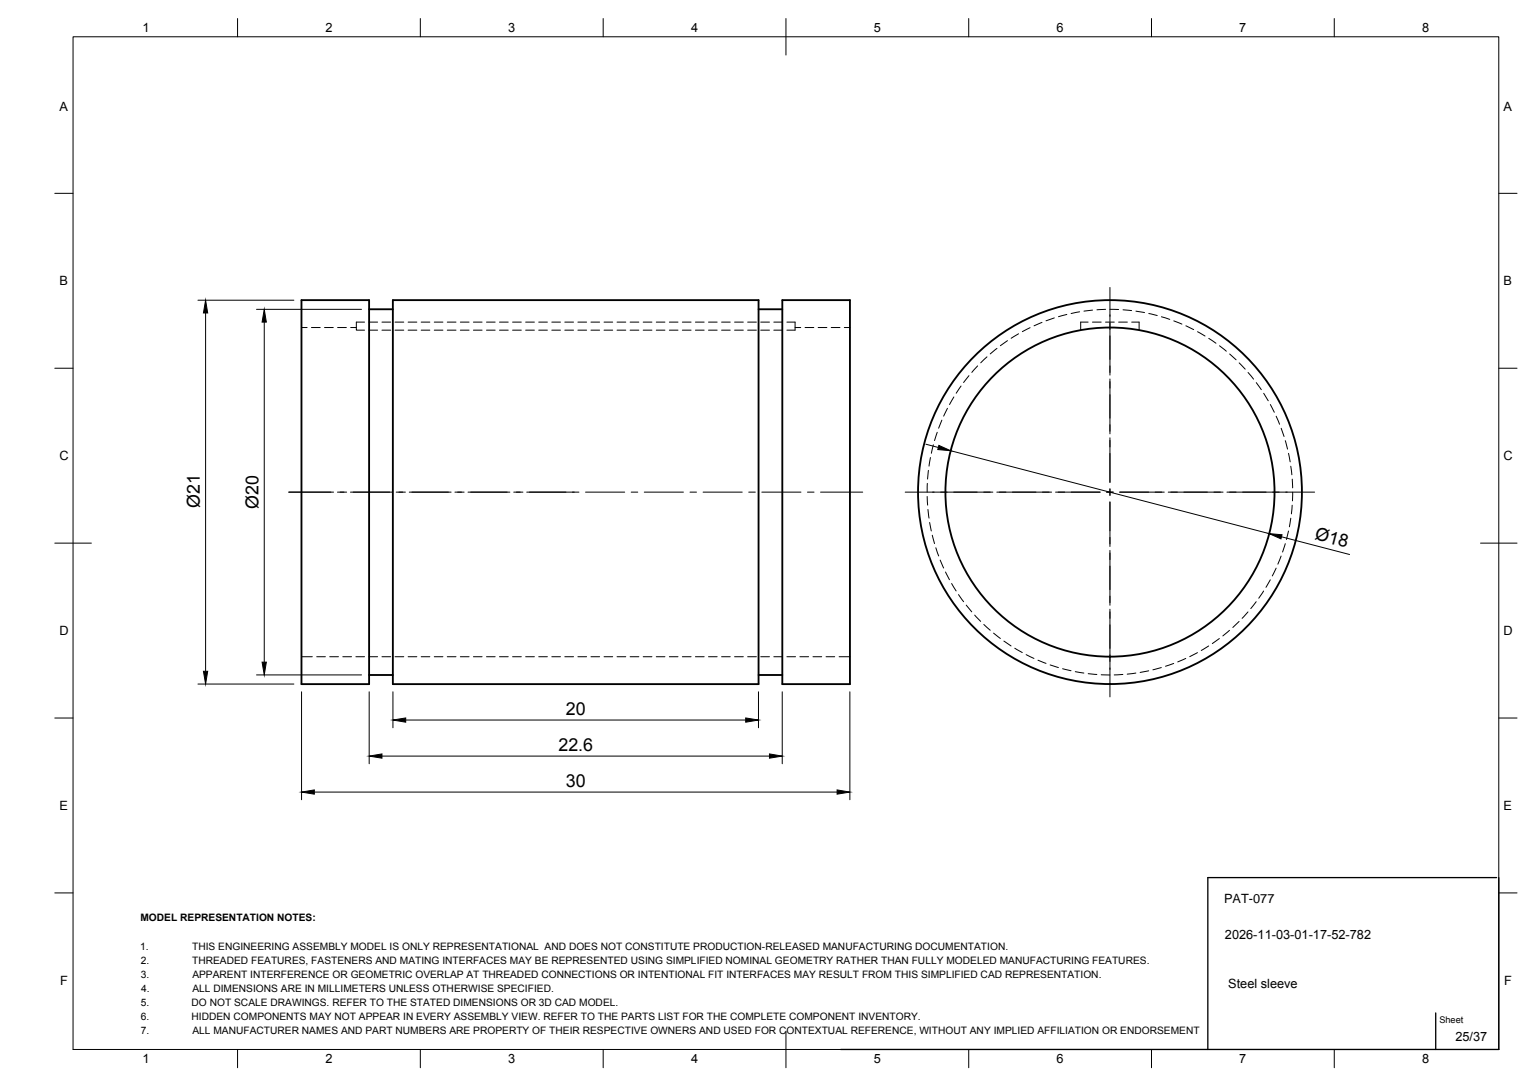
ISO-10303-21;
HEADER;
/* Generated by software containing ST-Developer
 * from STEP Tools, Inc. (www.steptools.com) 
 */

FILE_DESCRIPTION(
/* description */ ('Pallet stop with pneumatic fitting'),
/* implementation_level */ '2;1');

FILE_NAME(
/* name */ 'Steel sleeve.step',
/* time_stamp */ '2026-10-27T10:51:41-07:00',
/* author */ (''),
/* organization */ (''),
/* preprocessor_version */ 'ST-DEVELOPER v20.2',
/* originating_system */ 'Autodesk Translation Framework v15.17.0.0',
/* authorisation */ '');

FILE_SCHEMA (('AUTOMOTIVE_DESIGN { 1 0 10303 214 3 1 1 }'));
ENDSEC;

DATA;
#10=MECHANICAL_DESIGN_GEOMETRIC_PRESENTATION_REPRESENTATION('',(#375),#10265);
#311=SHAPE_REPRESENTATION_RELATIONSHIP('SRR','None',#10425,#343);
#343=ADVANCED_BREP_SHAPE_REPRESENTATION('',(#407),#10249);
#375=STYLED_ITEM('',(#10669),#407);
#407=MANIFOLD_SOLID_BREP('Body1',#5063);
#504=FACE_BOUND('',#1299,.T.);
#505=FACE_BOUND('',#1302,.T.);
#506=FACE_BOUND('',#1305,.T.);
#507=FACE_BOUND('',#1308,.T.);
#508=FACE_BOUND('',#1311,.T.);
#509=FACE_BOUND('',#1314,.T.);
#510=FACE_BOUND('',#1316,.T.);
#632=PLANE('',#5753);
#633=PLANE('',#5755);
#634=PLANE('',#5756);
#635=PLANE('',#5758);
#636=PLANE('',#5759);
#637=PLANE('',#5760);
#638=PLANE('',#5765);
#639=PLANE('',#5769);
#640=PLANE('',#5773);
#641=PLANE('',#5777);
#642=PLANE('',#5781);
#894=FACE_OUTER_BOUND('',#1293,.T.);
#895=FACE_OUTER_BOUND('',#1294,.T.);
#896=FACE_OUTER_BOUND('',#1295,.T.);
#897=FACE_OUTER_BOUND('',#1296,.T.);
#898=FACE_OUTER_BOUND('',#1297,.T.);
#899=FACE_OUTER_BOUND('',#1298,.T.);
#900=FACE_OUTER_BOUND('',#1300,.T.);
#901=FACE_OUTER_BOUND('',#1301,.T.);
#902=FACE_OUTER_BOUND('',#1303,.T.);
#903=FACE_OUTER_BOUND('',#1304,.T.);
#904=FACE_OUTER_BOUND('',#1306,.T.);
#905=FACE_OUTER_BOUND('',#1307,.T.);
#906=FACE_OUTER_BOUND('',#1309,.T.);
#907=FACE_OUTER_BOUND('',#1310,.T.);
#908=FACE_OUTER_BOUND('',#1312,.T.);
#909=FACE_OUTER_BOUND('',#1313,.T.);
#910=FACE_OUTER_BOUND('',#1315,.T.);
#1293=EDGE_LOOP('',(#4000,#4001,#4002,#4003));
#1294=EDGE_LOOP('',(#4004,#4005,#4006,#4007));
#1295=EDGE_LOOP('',(#4008,#4009,#4010,#4011));
#1296=EDGE_LOOP('',(#4012,#4013,#4014,#4015));
#1297=EDGE_LOOP('',(#4016,#4017,#4018,#4019));
#1298=EDGE_LOOP('',(#4020));
#1299=EDGE_LOOP('',(#4021));
#1300=EDGE_LOOP('',(#4022,#4023,#4024,#4025));
#1301=EDGE_LOOP('',(#4026));
#1302=EDGE_LOOP('',(#4027));
#1303=EDGE_LOOP('',(#4028,#4029,#4030,#4031));
#1304=EDGE_LOOP('',(#4032));
#1305=EDGE_LOOP('',(#4033));
#1306=EDGE_LOOP('',(#4034,#4035,#4036,#4037));
#1307=EDGE_LOOP('',(#4038));
#1308=EDGE_LOOP('',(#4039));
#1309=EDGE_LOOP('',(#4040,#4041,#4042,#4043));
#1310=EDGE_LOOP('',(#4044));
#1311=EDGE_LOOP('',(#4045));
#1312=EDGE_LOOP('',(#4046,#4047,#4048,#4049));
#1313=EDGE_LOOP('',(#4050));
#1314=EDGE_LOOP('',(#4051));
#1315=EDGE_LOOP('',(#4052,#4053,#4054,#4055));
#1316=EDGE_LOOP('',(#4056,#4057,#4058,#4059));
#1636=LINE('',#9366,#1971);
#1637=LINE('',#9368,#1972);
#1638=LINE('',#9369,#1973);
#1639=LINE('',#9372,#1974);
#1640=LINE('',#9374,#1975);
#1641=LINE('',#9375,#1976);
#1642=LINE('',#9380,#1977);
#1643=LINE('',#9381,#1978);
#1644=LINE('',#9383,#1979);
#1645=LINE('',#9384,#1980);
#1646=LINE('',#9394,#1981);
#1647=LINE('',#9401,#1982);
#1648=LINE('',#9408,#1983);
#1649=LINE('',#9415,#1984);
#1650=LINE('',#9422,#1985);
#1651=LINE('',#9427,#1986);
#1971=VECTOR('',#6881,1.);
#1972=VECTOR('',#6882,1.);
#1973=VECTOR('',#6883,1.);
#1974=VECTOR('',#6886,1.);
#1975=VECTOR('',#6887,1.);
#1976=VECTOR('',#6888,1.);
#1977=VECTOR('',#6893,1.);
#1978=VECTOR('',#6894,1.);
#1979=VECTOR('',#6897,1.);
#1980=VECTOR('',#6898,1.);
#1981=VECTOR('',#6911,1.05);
#1982=VECTOR('',#6920,1.);
#1983=VECTOR('',#6929,1.05);
#1984=VECTOR('',#6938,1.);
#1985=VECTOR('',#6947,1.05);
#1986=VECTOR('',#6954,0.9);
#2302=CIRCLE('',#5754,0.9);
#2303=CIRCLE('',#5757,0.9);
#2304=CIRCLE('',#5761,1.05);
#2305=CIRCLE('',#5762,0.9);
#2306=CIRCLE('',#5764,1.05);
#2307=CIRCLE('',#5766,1.);
#2308=CIRCLE('',#5768,1.);
#2309=CIRCLE('',#5770,1.05);
#2310=CIRCLE('',#5772,1.05);
#2311=CIRCLE('',#5774,1.);
#2312=CIRCLE('',#5776,1.);
#2313=CIRCLE('',#5778,1.05);
#2314=CIRCLE('',#5780,1.05);
#2315=CIRCLE('',#5782,0.9);
#2602=VERTEX_POINT('',#9362);
#2603=VERTEX_POINT('',#9363);
#2604=VERTEX_POINT('',#9365);
#2605=VERTEX_POINT('',#9367);
#2606=VERTEX_POINT('',#9371);
#2607=VERTEX_POINT('',#9373);
#2608=VERTEX_POINT('',#9377);
#2609=VERTEX_POINT('',#9379);
#2610=VERTEX_POINT('',#9387);
#2611=VERTEX_POINT('',#9389);
#2612=VERTEX_POINT('',#9392);
#2613=VERTEX_POINT('',#9396);
#2614=VERTEX_POINT('',#9399);
#2615=VERTEX_POINT('',#9403);
#2616=VERTEX_POINT('',#9406);
#2617=VERTEX_POINT('',#9410);
#2618=VERTEX_POINT('',#9413);
#2619=VERTEX_POINT('',#9417);
#2620=VERTEX_POINT('',#9420);
#2621=VERTEX_POINT('',#9424);
#3099=EDGE_CURVE('',#2602,#2603,#2302,.T.);
#3100=EDGE_CURVE('',#2604,#2602,#1636,.T.);
#3101=EDGE_CURVE('',#2605,#2604,#1637,.T.);
#3102=EDGE_CURVE('',#2603,#2605,#1638,.T.);
#3103=EDGE_CURVE('',#2603,#2606,#1639,.T.);
#3104=EDGE_CURVE('',#2607,#2605,#1640,.T.);
#3105=EDGE_CURVE('',#2607,#2606,#1641,.T.);
#3106=EDGE_CURVE('',#2606,#2608,#2303,.T.);
#3107=EDGE_CURVE('',#2609,#2607,#1642,.T.);
#3108=EDGE_CURVE('',#2608,#2609,#1643,.T.);
#3109=EDGE_CURVE('',#2608,#2602,#1644,.T.);
#3110=EDGE_CURVE('',#2609,#2604,#1645,.T.);
#3111=EDGE_CURVE('',#2610,#2610,#2304,.T.);
#3112=EDGE_CURVE('',#2611,#2611,#2305,.T.);
#3113=EDGE_CURVE('',#2612,#2612,#2306,.T.);
#3114=EDGE_CURVE('',#2612,#2610,#1646,.T.);
#3115=EDGE_CURVE('',#2613,#2613,#2307,.T.);
#3116=EDGE_CURVE('',#2614,#2614,#2308,.T.);
#3117=EDGE_CURVE('',#2614,#2613,#1647,.T.);
#3118=EDGE_CURVE('',#2615,#2615,#2309,.T.);
#3119=EDGE_CURVE('',#2616,#2616,#2310,.T.);
#3120=EDGE_CURVE('',#2616,#2615,#1648,.T.);
#3121=EDGE_CURVE('',#2617,#2617,#2311,.T.);
#3122=EDGE_CURVE('',#2618,#2618,#2312,.T.);
#3123=EDGE_CURVE('',#2618,#2617,#1649,.T.);
#3124=EDGE_CURVE('',#2619,#2619,#2313,.T.);
#3125=EDGE_CURVE('',#2620,#2620,#2314,.T.);
#3126=EDGE_CURVE('',#2620,#2619,#1650,.T.);
#3127=EDGE_CURVE('',#2621,#2621,#2315,.T.);
#3128=EDGE_CURVE('',#2621,#2611,#1651,.T.);
#4000=ORIENTED_EDGE('',*,*,#3099,.F.);
#4001=ORIENTED_EDGE('',*,*,#3100,.F.);
#4002=ORIENTED_EDGE('',*,*,#3101,.F.);
#4003=ORIENTED_EDGE('',*,*,#3102,.F.);
#4004=ORIENTED_EDGE('',*,*,#3103,.F.);
#4005=ORIENTED_EDGE('',*,*,#3102,.T.);
#4006=ORIENTED_EDGE('',*,*,#3104,.F.);
#4007=ORIENTED_EDGE('',*,*,#3105,.T.);
#4008=ORIENTED_EDGE('',*,*,#3106,.F.);
#4009=ORIENTED_EDGE('',*,*,#3105,.F.);
#4010=ORIENTED_EDGE('',*,*,#3107,.F.);
#4011=ORIENTED_EDGE('',*,*,#3108,.F.);
#4012=ORIENTED_EDGE('',*,*,#3109,.F.);
#4013=ORIENTED_EDGE('',*,*,#3108,.T.);
#4014=ORIENTED_EDGE('',*,*,#3110,.T.);
#4015=ORIENTED_EDGE('',*,*,#3100,.T.);
#4016=ORIENTED_EDGE('',*,*,#3110,.F.);
#4017=ORIENTED_EDGE('',*,*,#3107,.T.);
#4018=ORIENTED_EDGE('',*,*,#3104,.T.);
#4019=ORIENTED_EDGE('',*,*,#3101,.T.);
#4020=ORIENTED_EDGE('',*,*,#3111,.F.);
#4021=ORIENTED_EDGE('',*,*,#3112,.T.);
#4022=ORIENTED_EDGE('',*,*,#3113,.F.);
#4023=ORIENTED_EDGE('',*,*,#3114,.T.);
#4024=ORIENTED_EDGE('',*,*,#3111,.T.);
#4025=ORIENTED_EDGE('',*,*,#3114,.F.);
#4026=ORIENTED_EDGE('',*,*,#3113,.T.);
#4027=ORIENTED_EDGE('',*,*,#3115,.F.);
#4028=ORIENTED_EDGE('',*,*,#3116,.F.);
#4029=ORIENTED_EDGE('',*,*,#3117,.T.);
#4030=ORIENTED_EDGE('',*,*,#3115,.T.);
#4031=ORIENTED_EDGE('',*,*,#3117,.F.);
#4032=ORIENTED_EDGE('',*,*,#3118,.F.);
#4033=ORIENTED_EDGE('',*,*,#3116,.T.);
#4034=ORIENTED_EDGE('',*,*,#3119,.F.);
#4035=ORIENTED_EDGE('',*,*,#3120,.T.);
#4036=ORIENTED_EDGE('',*,*,#3118,.T.);
#4037=ORIENTED_EDGE('',*,*,#3120,.F.);
#4038=ORIENTED_EDGE('',*,*,#3119,.T.);
#4039=ORIENTED_EDGE('',*,*,#3121,.F.);
#4040=ORIENTED_EDGE('',*,*,#3122,.F.);
#4041=ORIENTED_EDGE('',*,*,#3123,.T.);
#4042=ORIENTED_EDGE('',*,*,#3121,.T.);
#4043=ORIENTED_EDGE('',*,*,#3123,.F.);
#4044=ORIENTED_EDGE('',*,*,#3124,.F.);
#4045=ORIENTED_EDGE('',*,*,#3122,.T.);
#4046=ORIENTED_EDGE('',*,*,#3125,.F.);
#4047=ORIENTED_EDGE('',*,*,#3126,.T.);
#4048=ORIENTED_EDGE('',*,*,#3124,.T.);
#4049=ORIENTED_EDGE('',*,*,#3126,.F.);
#4050=ORIENTED_EDGE('',*,*,#3125,.T.);
#4051=ORIENTED_EDGE('',*,*,#3127,.F.);
#4052=ORIENTED_EDGE('',*,*,#3127,.T.);
#4053=ORIENTED_EDGE('',*,*,#3128,.T.);
#4054=ORIENTED_EDGE('',*,*,#3112,.F.);
#4055=ORIENTED_EDGE('',*,*,#3128,.F.);
#4056=ORIENTED_EDGE('',*,*,#3106,.T.);
#4057=ORIENTED_EDGE('',*,*,#3109,.T.);
#4058=ORIENTED_EDGE('',*,*,#3099,.T.);
#4059=ORIENTED_EDGE('',*,*,#3103,.T.);
#4692=CYLINDRICAL_SURFACE('',#5763,1.05);
#4693=CYLINDRICAL_SURFACE('',#5767,1.);
#4694=CYLINDRICAL_SURFACE('',#5771,1.05);
#4695=CYLINDRICAL_SURFACE('',#5775,1.);
#4696=CYLINDRICAL_SURFACE('',#5779,1.05);
#4697=CYLINDRICAL_SURFACE('',#5783,0.9);
#4889=ADVANCED_FACE('',(#894),#632,.F.);
#4890=ADVANCED_FACE('',(#895),#633,.F.);
#4891=ADVANCED_FACE('',(#896),#634,.F.);
#4892=ADVANCED_FACE('',(#897),#635,.F.);
#4893=ADVANCED_FACE('',(#898),#636,.F.);
#4894=ADVANCED_FACE('',(#899,#504),#637,.T.);
#4895=ADVANCED_FACE('',(#900),#4692,.T.);
#4896=ADVANCED_FACE('',(#901,#505),#638,.T.);
#4897=ADVANCED_FACE('',(#902),#4693,.T.);
#4898=ADVANCED_FACE('',(#903,#506),#639,.T.);
#4899=ADVANCED_FACE('',(#904),#4694,.T.);
#4900=ADVANCED_FACE('',(#905,#507),#640,.T.);
#4901=ADVANCED_FACE('',(#906),#4695,.T.);
#4902=ADVANCED_FACE('',(#907,#508),#641,.T.);
#4903=ADVANCED_FACE('',(#908),#4696,.T.);
#4904=ADVANCED_FACE('',(#909,#509),#642,.T.);
#4905=ADVANCED_FACE('',(#910,#510),#4697,.F.);
#5063=CLOSED_SHELL('',(#4889,#4890,#4891,#4892,#4893,#4894,#4895,#4896,
#4897,#4898,#4899,#4900,#4901,#4902,#4903,#4904,#4905));
#5752=AXIS2_PLACEMENT_3D('',#9360,#6875,#6876);
#5753=AXIS2_PLACEMENT_3D('',#9361,#6877,#6878);
#5754=AXIS2_PLACEMENT_3D('',#9364,#6879,#6880);
#5755=AXIS2_PLACEMENT_3D('',#9370,#6884,#6885);
#5756=AXIS2_PLACEMENT_3D('',#9376,#6889,#6890);
#5757=AXIS2_PLACEMENT_3D('',#9378,#6891,#6892);
#5758=AXIS2_PLACEMENT_3D('',#9382,#6895,#6896);
#5759=AXIS2_PLACEMENT_3D('',#9385,#6899,#6900);
#5760=AXIS2_PLACEMENT_3D('',#9386,#6901,#6902);
#5761=AXIS2_PLACEMENT_3D('',#9388,#6903,#6904);
#5762=AXIS2_PLACEMENT_3D('',#9390,#6905,#6906);
#5763=AXIS2_PLACEMENT_3D('',#9391,#6907,#6908);
#5764=AXIS2_PLACEMENT_3D('',#9393,#6909,#6910);
#5765=AXIS2_PLACEMENT_3D('',#9395,#6912,#6913);
#5766=AXIS2_PLACEMENT_3D('',#9397,#6914,#6915);
#5767=AXIS2_PLACEMENT_3D('',#9398,#6916,#6917);
#5768=AXIS2_PLACEMENT_3D('',#9400,#6918,#6919);
#5769=AXIS2_PLACEMENT_3D('',#9402,#6921,#6922);
#5770=AXIS2_PLACEMENT_3D('',#9404,#6923,#6924);
#5771=AXIS2_PLACEMENT_3D('',#9405,#6925,#6926);
#5772=AXIS2_PLACEMENT_3D('',#9407,#6927,#6928);
#5773=AXIS2_PLACEMENT_3D('',#9409,#6930,#6931);
#5774=AXIS2_PLACEMENT_3D('',#9411,#6932,#6933);
#5775=AXIS2_PLACEMENT_3D('',#9412,#6934,#6935);
#5776=AXIS2_PLACEMENT_3D('',#9414,#6936,#6937);
#5777=AXIS2_PLACEMENT_3D('',#9416,#6939,#6940);
#5778=AXIS2_PLACEMENT_3D('',#9418,#6941,#6942);
#5779=AXIS2_PLACEMENT_3D('',#9419,#6943,#6944);
#5780=AXIS2_PLACEMENT_3D('',#9421,#6945,#6946);
#5781=AXIS2_PLACEMENT_3D('',#9423,#6948,#6949);
#5782=AXIS2_PLACEMENT_3D('',#9425,#6950,#6951);
#5783=AXIS2_PLACEMENT_3D('',#9426,#6952,#6953);
#6875=DIRECTION('axis',(0.,0.,1.));
#6876=DIRECTION('refdir',(1.,0.,0.));
#6877=DIRECTION('center_axis',(0.,1.,0.));
#6878=DIRECTION('ref_axis',(0.,0.,1.));
#6879=DIRECTION('center_axis',(0.,-1.,0.));
#6880=DIRECTION('ref_axis',(1.,0.,0.));
#6881=DIRECTION('',(-1.,0.,0.));
#6882=DIRECTION('',(0.,0.,-1.));
#6883=DIRECTION('',(1.,0.,0.));
#6884=DIRECTION('center_axis',(0.,0.,1.));
#6885=DIRECTION('ref_axis',(1.,0.,0.));
#6886=DIRECTION('',(0.,-1.,0.));
#6887=DIRECTION('',(0.,1.,0.));
#6888=DIRECTION('',(-1.,0.,0.));
#6889=DIRECTION('center_axis',(0.,-1.,0.));
#6890=DIRECTION('ref_axis',(0.,0.,-1.));
#6891=DIRECTION('center_axis',(0.,1.,0.));
#6892=DIRECTION('ref_axis',(1.,0.,0.));
#6893=DIRECTION('',(0.,0.,1.));
#6894=DIRECTION('',(1.,0.,0.));
#6895=DIRECTION('center_axis',(0.,0.,-1.));
#6896=DIRECTION('ref_axis',(-1.,0.,0.));
#6897=DIRECTION('',(0.,1.,0.));
#6898=DIRECTION('',(0.,1.,0.));
#6899=DIRECTION('center_axis',(1.,0.,0.));
#6900=DIRECTION('ref_axis',(0.,0.,-1.));
#6901=DIRECTION('center_axis',(0.,1.,0.));
#6902=DIRECTION('ref_axis',(0.,0.,1.));
#6903=DIRECTION('center_axis',(0.,-1.,0.));
#6904=DIRECTION('ref_axis',(1.,0.,0.));
#6905=DIRECTION('center_axis',(0.,-1.,0.));
#6906=DIRECTION('ref_axis',(1.,0.,0.));
#6907=DIRECTION('center_axis',(0.,-1.,0.));
#6908=DIRECTION('ref_axis',(1.,0.,0.));
#6909=DIRECTION('center_axis',(0.,-1.,0.));
#6910=DIRECTION('ref_axis',(1.,0.,0.));
#6911=DIRECTION('',(0.,1.,0.));
#6912=DIRECTION('center_axis',(0.,-1.,0.));
#6913=DIRECTION('ref_axis',(0.,0.,-1.));
#6914=DIRECTION('center_axis',(0.,-1.,0.));
#6915=DIRECTION('ref_axis',(1.,0.,0.));
#6916=DIRECTION('center_axis',(0.,-1.,0.));
#6917=DIRECTION('ref_axis',(1.,0.,0.));
#6918=DIRECTION('center_axis',(0.,-1.,0.));
#6919=DIRECTION('ref_axis',(1.,0.,0.));
#6920=DIRECTION('',(0.,1.,0.));
#6921=DIRECTION('center_axis',(0.,1.,0.));
#6922=DIRECTION('ref_axis',(0.,0.,1.));
#6923=DIRECTION('center_axis',(0.,-1.,0.));
#6924=DIRECTION('ref_axis',(1.,0.,0.));
#6925=DIRECTION('center_axis',(0.,-1.,0.));
#6926=DIRECTION('ref_axis',(1.,0.,0.));
#6927=DIRECTION('center_axis',(0.,-1.,0.));
#6928=DIRECTION('ref_axis',(1.,0.,0.));
#6929=DIRECTION('',(0.,1.,0.));
#6930=DIRECTION('center_axis',(0.,-1.,0.));
#6931=DIRECTION('ref_axis',(0.,0.,-1.));
#6932=DIRECTION('center_axis',(0.,-1.,0.));
#6933=DIRECTION('ref_axis',(1.,0.,0.));
#6934=DIRECTION('center_axis',(0.,-1.,0.));
#6935=DIRECTION('ref_axis',(1.,0.,0.));
#6936=DIRECTION('center_axis',(0.,-1.,0.));
#6937=DIRECTION('ref_axis',(1.,0.,0.));
#6938=DIRECTION('',(0.,1.,0.));
#6939=DIRECTION('center_axis',(0.,1.,0.));
#6940=DIRECTION('ref_axis',(0.,0.,1.));
#6941=DIRECTION('center_axis',(0.,-1.,0.));
#6942=DIRECTION('ref_axis',(1.,0.,0.));
#6943=DIRECTION('center_axis',(0.,-1.,0.));
#6944=DIRECTION('ref_axis',(1.,0.,0.));
#6945=DIRECTION('center_axis',(0.,-1.,0.));
#6946=DIRECTION('ref_axis',(1.,0.,0.));
#6947=DIRECTION('',(0.,1.,0.));
#6948=DIRECTION('center_axis',(0.,-1.,0.));
#6949=DIRECTION('ref_axis',(0.,0.,-1.));
#6950=DIRECTION('center_axis',(0.,-1.,0.));
#6951=DIRECTION('ref_axis',(1.,0.,0.));
#6952=DIRECTION('center_axis',(0.,-1.,0.));
#6953=DIRECTION('ref_axis',(1.,0.,0.));
#6954=DIRECTION('',(0.,1.,0.));
#9360=CARTESIAN_POINT('',(0.,0.,0.));
#9361=CARTESIAN_POINT('Origin',(0.75,1.2,0.));
#9362=CARTESIAN_POINT('',(0.885663593019381,1.2,-0.16));
#9363=CARTESIAN_POINT('',(0.885663593019381,1.2,0.16));
#9364=CARTESIAN_POINT('Origin',(0.,1.2,0.));
#9365=CARTESIAN_POINT('',(0.93,1.2,-0.16));
#9366=CARTESIAN_POINT('',(0.93,1.2,-0.16));
#9367=CARTESIAN_POINT('',(0.93,1.2,0.16));
#9368=CARTESIAN_POINT('',(0.93,1.2,0.16));
#9369=CARTESIAN_POINT('',(0.57,1.2,0.16));
#9370=CARTESIAN_POINT('Origin',(0.57,0.,0.16));
#9371=CARTESIAN_POINT('',(0.885663593019381,-1.2,0.16));
#9372=CARTESIAN_POINT('',(0.885663593019381,0.,0.16));
#9373=CARTESIAN_POINT('',(0.93,-1.2,0.16));
#9374=CARTESIAN_POINT('',(0.93,0.,0.16));
#9375=CARTESIAN_POINT('',(0.57,-1.2,0.16));
#9376=CARTESIAN_POINT('Origin',(0.75,-1.2,0.));
#9377=CARTESIAN_POINT('',(0.885663593019381,-1.2,-0.16));
#9378=CARTESIAN_POINT('Origin',(0.,-1.2,0.));
#9379=CARTESIAN_POINT('',(0.93,-1.2,-0.16));
#9380=CARTESIAN_POINT('',(0.93,-1.2,0.16));
#9381=CARTESIAN_POINT('',(0.93,-1.2,-0.16));
#9382=CARTESIAN_POINT('Origin',(0.93,0.,-0.16));
#9383=CARTESIAN_POINT('',(0.885663593019381,0.,-0.16));
#9384=CARTESIAN_POINT('',(0.93,0.,-0.16));
#9385=CARTESIAN_POINT('Origin',(0.93,0.,0.16));
#9386=CARTESIAN_POINT('Origin',(1.05,1.5,0.));
#9387=CARTESIAN_POINT('',(-1.05,1.5,-1.28587913910472E-16));
#9388=CARTESIAN_POINT('Origin',(0.,1.5,0.));
#9389=CARTESIAN_POINT('',(-0.9,1.5,-1.10218211923262E-16));
#9390=CARTESIAN_POINT('Origin',(0.,1.5,0.));
#9391=CARTESIAN_POINT('Origin',(0.,1.315,0.));
#9392=CARTESIAN_POINT('',(-1.05,1.13,-1.28587913910472E-16));
#9393=CARTESIAN_POINT('Origin',(0.,1.13,0.));
#9394=CARTESIAN_POINT('',(-1.05,1.315,-1.28587913910472E-16));
#9395=CARTESIAN_POINT('Origin',(1.,1.13,0.));
#9396=CARTESIAN_POINT('',(-1.,1.13,-1.22464679914735E-16));
#9397=CARTESIAN_POINT('Origin',(0.,1.13,0.));
#9398=CARTESIAN_POINT('Origin',(0.,1.065,0.));
#9399=CARTESIAN_POINT('',(-1.,1.,-1.22464679914735E-16));
#9400=CARTESIAN_POINT('Origin',(0.,1.,0.));
#9401=CARTESIAN_POINT('',(-1.,1.065,-1.22464679914735E-16));
#9402=CARTESIAN_POINT('Origin',(1.05,1.,0.));
#9403=CARTESIAN_POINT('',(-1.05,1.,-1.28587913910472E-16));
#9404=CARTESIAN_POINT('Origin',(0.,1.,0.));
#9405=CARTESIAN_POINT('Origin',(0.,0.,0.));
#9406=CARTESIAN_POINT('',(-1.05,-1.,-1.28587913910472E-16));
#9407=CARTESIAN_POINT('Origin',(0.,-1.,0.));
#9408=CARTESIAN_POINT('',(-1.05,0.,-1.28587913910472E-16));
#9409=CARTESIAN_POINT('Origin',(1.,-1.,0.));
#9410=CARTESIAN_POINT('',(-1.,-1.,-1.22464679914735E-16));
#9411=CARTESIAN_POINT('Origin',(0.,-1.,0.));
#9412=CARTESIAN_POINT('Origin',(0.,-1.065,0.));
#9413=CARTESIAN_POINT('',(-1.,-1.13,-1.22464679914735E-16));
#9414=CARTESIAN_POINT('Origin',(0.,-1.13,0.));
#9415=CARTESIAN_POINT('',(-1.,-1.065,-1.22464679914735E-16));
#9416=CARTESIAN_POINT('Origin',(1.05,-1.13,0.));
#9417=CARTESIAN_POINT('',(-1.05,-1.13,-1.28587913910472E-16));
#9418=CARTESIAN_POINT('Origin',(0.,-1.13,0.));
#9419=CARTESIAN_POINT('Origin',(0.,-1.315,0.));
#9420=CARTESIAN_POINT('',(-1.05,-1.5,-1.28587913910472E-16));
#9421=CARTESIAN_POINT('Origin',(0.,-1.5,0.));
#9422=CARTESIAN_POINT('',(-1.05,-1.315,-1.28587913910472E-16));
#9423=CARTESIAN_POINT('Origin',(0.9,-1.5,0.));
#9424=CARTESIAN_POINT('',(-0.9,-1.5,-1.10218211923262E-16));
#9425=CARTESIAN_POINT('Origin',(0.,-1.5,0.));
#9426=CARTESIAN_POINT('Origin',(0.,0.,0.));
#9427=CARTESIAN_POINT('',(-0.9,0.,-1.10218211923262E-16));
#10211=UNCERTAINTY_MEASURE_WITH_UNIT(LENGTH_MEASURE(0.001),#10266,
'DISTANCE_ACCURACY_VALUE',
'Maximum model space distance between geometric entities at asserted c
onnectivities');
#10227=UNCERTAINTY_MEASURE_WITH_UNIT(LENGTH_MEASURE(0.001),#10266,
'DISTANCE_ACCURACY_VALUE',
'Maximum model space distance between geometric entities at asserted c
onnectivities');
#10249=(
GEOMETRIC_REPRESENTATION_CONTEXT(3)
GLOBAL_UNCERTAINTY_ASSIGNED_CONTEXT((#10211))
GLOBAL_UNIT_ASSIGNED_CONTEXT((#10266,#10268,#10269))
REPRESENTATION_CONTEXT('','3D')
);
#10265=(
GEOMETRIC_REPRESENTATION_CONTEXT(3)
GLOBAL_UNCERTAINTY_ASSIGNED_CONTEXT((#10227))
GLOBAL_UNIT_ASSIGNED_CONTEXT((#10266,#10268,#10269))
REPRESENTATION_CONTEXT('','3D')
);
#10266=(
LENGTH_UNIT()
NAMED_UNIT(*)
SI_UNIT(.CENTI.,.METRE.)
);
#10268=(
NAMED_UNIT(*)
PLANE_ANGLE_UNIT()
SI_UNIT($,.RADIAN.)
);
#10269=(
NAMED_UNIT(*)
SI_UNIT($,.STERADIAN.)
SOLID_ANGLE_UNIT()
);
#10291=SHAPE_DEFINITION_REPRESENTATION(#10328,#10425);
#10328=PRODUCT_DEFINITION_SHAPE('',$,#10463);
#10425=SHAPE_REPRESENTATION('',(#5752),#10249);
#10441=PRODUCT_DEFINITION_CONTEXT('part definition',#10554,'design');
#10463=PRODUCT_DEFINITION('Steel sleeve','Steel sleeve',#10500,#10441);
#10500=PRODUCT_DEFINITION_FORMATION('',$,#10577);
#10554=APPLICATION_CONTEXT(
'Core Data for Automotive Mechanical Design Process');
#10555=PRODUCT_CONTEXT('part definition',#10554,'mechanical');
#10577=PRODUCT('Steel sleeve','Steel sleeve','Steel sleeve',(#10555));
#10663=COLOUR_RGB('Off White',0.89,0.88,0.83);
#10664=FILL_AREA_STYLE_COLOUR('',#10663);
#10665=FILL_AREA_STYLE('',(#10664));
#10666=SURFACE_STYLE_FILL_AREA(#10665);
#10667=SURFACE_SIDE_STYLE('',(#10666));
#10668=SURFACE_STYLE_USAGE(.BOTH.,#10667);
#10669=PRESENTATION_STYLE_ASSIGNMENT((#10668));
ENDSEC;
END-ISO-10303-21;
